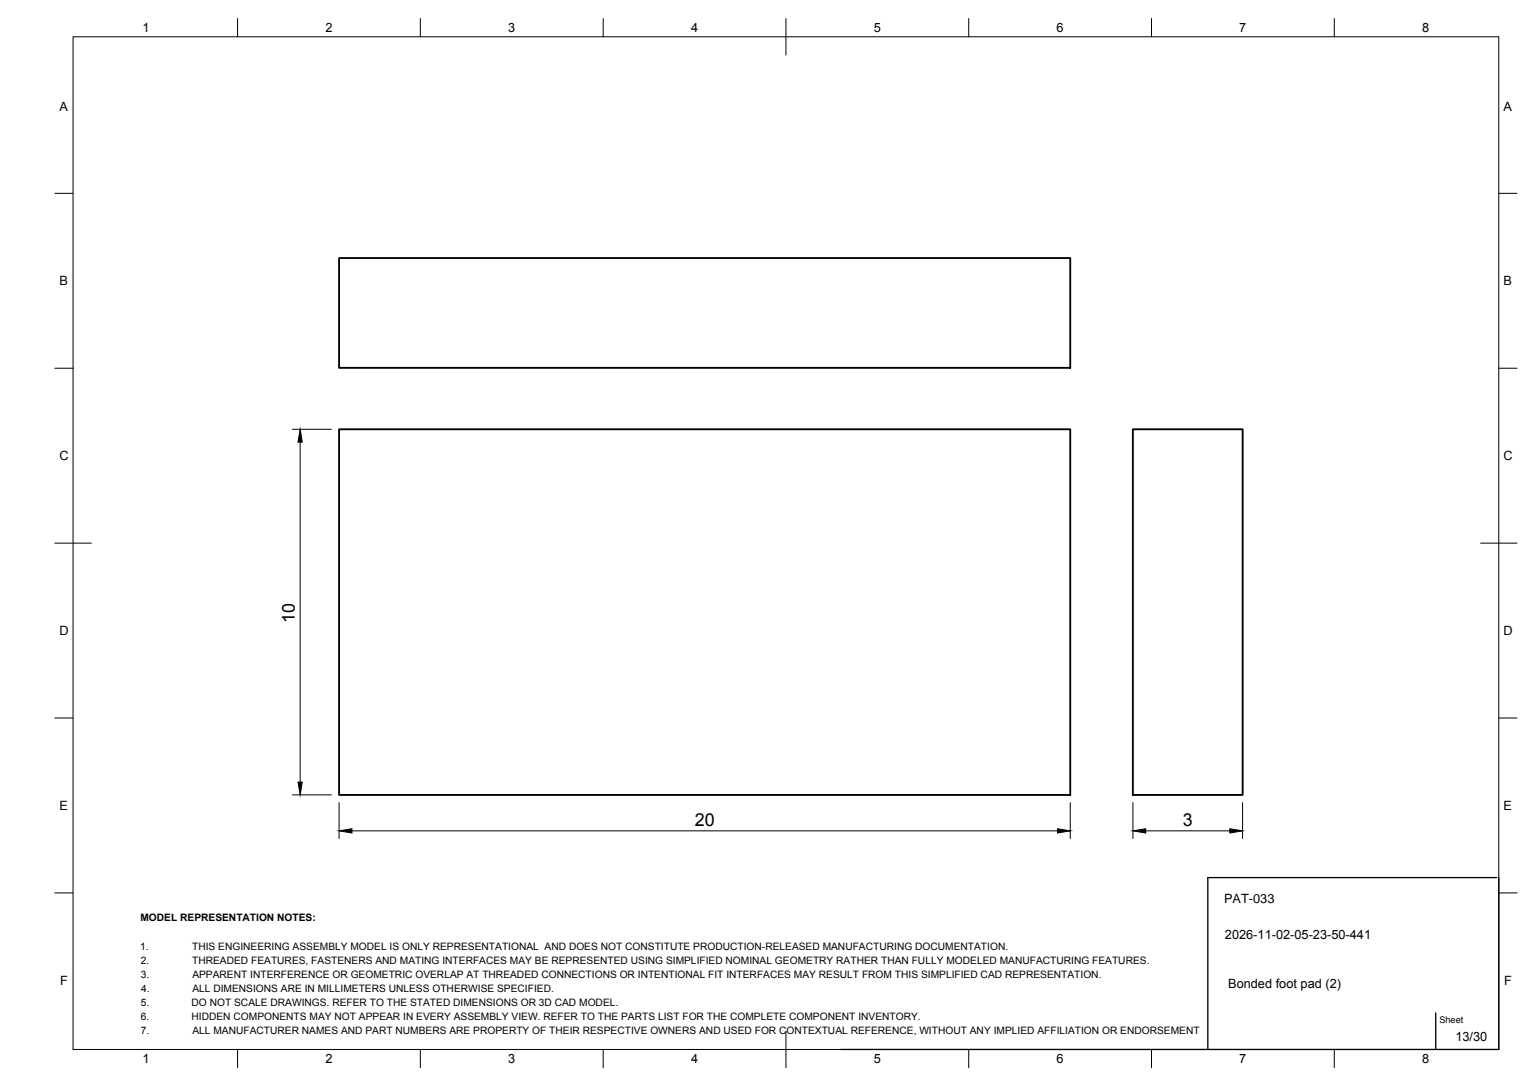
ISO-10303-21;
HEADER;
/* Generated by software containing ST-Developer
 * from STEP Tools, Inc. (www.steptools.com) 
 */

FILE_DESCRIPTION(
/* description */ ('Dual-rail gantry carriage'),
/* implementation_level */ '2;1');

FILE_NAME(
/* name */ 'Bonded foot pad (2).step',
/* time_stamp */ '2026-10-27T10:49:15-07:00',
/* author */ (''),
/* organization */ (''),
/* preprocessor_version */ 'ST-DEVELOPER v20.2',
/* originating_system */ 'Autodesk Translation Framework v15.17.0.0',
/* authorisation */ '');

FILE_SCHEMA (('AUTOMOTIVE_DESIGN { 1 0 10303 214 3 1 1 }'));
ENDSEC;

DATA;
#10=MECHANICAL_DESIGN_GEOMETRIC_PRESENTATION_REPRESENTATION('',(#593),#12804);
#531=SHAPE_REPRESENTATION_RELATIONSHIP('SRR','None',#13009,#562);
#562=ADVANCED_BREP_SHAPE_REPRESENTATION('',(#624),#12779);
#593=STYLED_ITEM('',(#13240),#624);
#624=MANIFOLD_SOLID_BREP('Body1',#7371);
#812=PLANE('',#7860);
#813=PLANE('',#7861);
#814=PLANE('',#7862);
#815=PLANE('',#7863);
#816=PLANE('',#7864);
#817=PLANE('',#7865);
#1116=FACE_OUTER_BOUND('',#1545,.T.);
#1117=FACE_OUTER_BOUND('',#1546,.T.);
#1118=FACE_OUTER_BOUND('',#1547,.T.);
#1119=FACE_OUTER_BOUND('',#1548,.T.);
#1120=FACE_OUTER_BOUND('',#1549,.T.);
#1121=FACE_OUTER_BOUND('',#1550,.T.);
#1545=EDGE_LOOP('',(#5379,#5380,#5381,#5382));
#1546=EDGE_LOOP('',(#5383,#5384,#5385,#5386));
#1547=EDGE_LOOP('',(#5387,#5388,#5389,#5390));
#1548=EDGE_LOOP('',(#5391,#5392,#5393,#5394));
#1549=EDGE_LOOP('',(#5395,#5396,#5397,#5398));
#1550=EDGE_LOOP('',(#5399,#5400,#5401,#5402));
#2064=LINE('',#11030,#2773);
#2065=LINE('',#11032,#2774);
#2066=LINE('',#11034,#2775);
#2067=LINE('',#11035,#2776);
#2068=LINE('',#11038,#2777);
#2069=LINE('',#11040,#2778);
#2070=LINE('',#11041,#2779);
#2071=LINE('',#11044,#2780);
#2072=LINE('',#11046,#2781);
#2073=LINE('',#11047,#2782);
#2074=LINE('',#11049,#2783);
#2075=LINE('',#11050,#2784);
#2773=VECTOR('',#8843,1.);
#2774=VECTOR('',#8844,1.);
#2775=VECTOR('',#8845,1.);
#2776=VECTOR('',#8846,1.);
#2777=VECTOR('',#8849,1.);
#2778=VECTOR('',#8850,1.);
#2779=VECTOR('',#8851,1.);
#2780=VECTOR('',#8854,1.);
#2781=VECTOR('',#8855,1.);
#2782=VECTOR('',#8856,1.);
#2783=VECTOR('',#8859,1.);
#2784=VECTOR('',#8860,1.);
#3670=VERTEX_POINT('',#11028);
#3671=VERTEX_POINT('',#11029);
#3672=VERTEX_POINT('',#11031);
#3673=VERTEX_POINT('',#11033);
#3674=VERTEX_POINT('',#11037);
#3675=VERTEX_POINT('',#11039);
#3676=VERTEX_POINT('',#11043);
#3677=VERTEX_POINT('',#11045);
#4312=EDGE_CURVE('',#3670,#3671,#2064,.T.);
#4313=EDGE_CURVE('',#3671,#3672,#2065,.T.);
#4314=EDGE_CURVE('',#3673,#3672,#2066,.T.);
#4315=EDGE_CURVE('',#3670,#3673,#2067,.T.);
#4316=EDGE_CURVE('',#3674,#3670,#2068,.T.);
#4317=EDGE_CURVE('',#3675,#3673,#2069,.T.);
#4318=EDGE_CURVE('',#3674,#3675,#2070,.T.);
#4319=EDGE_CURVE('',#3676,#3674,#2071,.T.);
#4320=EDGE_CURVE('',#3677,#3675,#2072,.T.);
#4321=EDGE_CURVE('',#3676,#3677,#2073,.T.);
#4322=EDGE_CURVE('',#3671,#3676,#2074,.T.);
#4323=EDGE_CURVE('',#3672,#3677,#2075,.T.);
#5379=ORIENTED_EDGE('',*,*,#4312,.T.);
#5380=ORIENTED_EDGE('',*,*,#4313,.T.);
#5381=ORIENTED_EDGE('',*,*,#4314,.F.);
#5382=ORIENTED_EDGE('',*,*,#4315,.F.);
#5383=ORIENTED_EDGE('',*,*,#4316,.T.);
#5384=ORIENTED_EDGE('',*,*,#4315,.T.);
#5385=ORIENTED_EDGE('',*,*,#4317,.F.);
#5386=ORIENTED_EDGE('',*,*,#4318,.F.);
#5387=ORIENTED_EDGE('',*,*,#4319,.T.);
#5388=ORIENTED_EDGE('',*,*,#4318,.T.);
#5389=ORIENTED_EDGE('',*,*,#4320,.F.);
#5390=ORIENTED_EDGE('',*,*,#4321,.F.);
#5391=ORIENTED_EDGE('',*,*,#4322,.T.);
#5392=ORIENTED_EDGE('',*,*,#4321,.T.);
#5393=ORIENTED_EDGE('',*,*,#4323,.F.);
#5394=ORIENTED_EDGE('',*,*,#4313,.F.);
#5395=ORIENTED_EDGE('',*,*,#4323,.T.);
#5396=ORIENTED_EDGE('',*,*,#4320,.T.);
#5397=ORIENTED_EDGE('',*,*,#4317,.T.);
#5398=ORIENTED_EDGE('',*,*,#4314,.T.);
#5399=ORIENTED_EDGE('',*,*,#4322,.F.);
#5400=ORIENTED_EDGE('',*,*,#4312,.F.);
#5401=ORIENTED_EDGE('',*,*,#4316,.F.);
#5402=ORIENTED_EDGE('',*,*,#4319,.F.);
#7042=ADVANCED_FACE('',(#1116),#812,.T.);
#7043=ADVANCED_FACE('',(#1117),#813,.T.);
#7044=ADVANCED_FACE('',(#1118),#814,.T.);
#7045=ADVANCED_FACE('',(#1119),#815,.T.);
#7046=ADVANCED_FACE('',(#1120),#816,.T.);
#7047=ADVANCED_FACE('',(#1121),#817,.F.);
#7371=CLOSED_SHELL('',(#7042,#7043,#7044,#7045,#7046,#7047));
#7859=AXIS2_PLACEMENT_3D('',#11026,#8839,#8840);
#7860=AXIS2_PLACEMENT_3D('',#11027,#8841,#8842);
#7861=AXIS2_PLACEMENT_3D('',#11036,#8847,#8848);
#7862=AXIS2_PLACEMENT_3D('',#11042,#8852,#8853);
#7863=AXIS2_PLACEMENT_3D('',#11048,#8857,#8858);
#7864=AXIS2_PLACEMENT_3D('',#11051,#8861,#8862);
#7865=AXIS2_PLACEMENT_3D('',#11052,#8863,#8864);
#8839=DIRECTION('axis',(0.,0.,1.));
#8840=DIRECTION('refdir',(1.,0.,0.));
#8841=DIRECTION('center_axis',(0.,1.,0.));
#8842=DIRECTION('ref_axis',(-1.,0.,0.));
#8843=DIRECTION('',(-1.,0.,0.));
#8844=DIRECTION('',(0.,0.,1.));
#8845=DIRECTION('',(-1.,0.,0.));
#8846=DIRECTION('',(0.,0.,1.));
#8847=DIRECTION('center_axis',(1.,0.,0.));
#8848=DIRECTION('ref_axis',(0.,1.,0.));
#8849=DIRECTION('',(0.,1.,0.));
#8850=DIRECTION('',(0.,1.,0.));
#8851=DIRECTION('',(0.,0.,1.));
#8852=DIRECTION('center_axis',(0.,-1.,0.));
#8853=DIRECTION('ref_axis',(1.,0.,0.));
#8854=DIRECTION('',(1.,0.,0.));
#8855=DIRECTION('',(1.,0.,0.));
#8856=DIRECTION('',(0.,0.,1.));
#8857=DIRECTION('center_axis',(-1.,0.,0.));
#8858=DIRECTION('ref_axis',(0.,-1.,0.));
#8859=DIRECTION('',(0.,-1.,0.));
#8860=DIRECTION('',(0.,-1.,0.));
#8861=DIRECTION('center_axis',(0.,0.,1.));
#8862=DIRECTION('ref_axis',(1.,0.,0.));
#8863=DIRECTION('center_axis',(0.,0.,1.));
#8864=DIRECTION('ref_axis',(1.,0.,0.));
#11026=CARTESIAN_POINT('',(0.,0.,0.));
#11027=CARTESIAN_POINT('Origin',(40.,-11.5,-1.1));
#11028=CARTESIAN_POINT('',(40.,-11.5,-1.1));
#11029=CARTESIAN_POINT('',(38.,-11.5,-1.1));
#11030=CARTESIAN_POINT('',(40.,-11.5,-1.1));
#11031=CARTESIAN_POINT('',(38.,-11.5,-0.8));
#11032=CARTESIAN_POINT('',(38.,-11.5,-1.1));
#11033=CARTESIAN_POINT('',(40.,-11.5,-0.8));
#11034=CARTESIAN_POINT('',(40.,-11.5,-0.8));
#11035=CARTESIAN_POINT('',(40.,-11.5,-1.1));
#11036=CARTESIAN_POINT('Origin',(40.,-12.5,-1.1));
#11037=CARTESIAN_POINT('',(40.,-12.5,-1.1));
#11038=CARTESIAN_POINT('',(40.,-12.5,-1.1));
#11039=CARTESIAN_POINT('',(40.,-12.5,-0.8));
#11040=CARTESIAN_POINT('',(40.,-12.5,-0.8));
#11041=CARTESIAN_POINT('',(40.,-12.5,-1.1));
#11042=CARTESIAN_POINT('Origin',(38.,-12.5,-1.1));
#11043=CARTESIAN_POINT('',(38.,-12.5,-1.1));
#11044=CARTESIAN_POINT('',(38.,-12.5,-1.1));
#11045=CARTESIAN_POINT('',(38.,-12.5,-0.8));
#11046=CARTESIAN_POINT('',(38.,-12.5,-0.8));
#11047=CARTESIAN_POINT('',(38.,-12.5,-1.1));
#11048=CARTESIAN_POINT('Origin',(38.,-11.5,-1.1));
#11049=CARTESIAN_POINT('',(38.,-11.5,-1.1));
#11050=CARTESIAN_POINT('',(38.,-11.5,-0.8));
#11051=CARTESIAN_POINT('Origin',(39.,-12.,-0.8));
#11052=CARTESIAN_POINT('Origin',(39.,-12.,-1.1));
#12743=UNCERTAINTY_MEASURE_WITH_UNIT(LENGTH_MEASURE(0.001),#12805,
'DISTANCE_ACCURACY_VALUE',
'Maximum model space distance between geometric entities at asserted c
onnectivities');
#12768=UNCERTAINTY_MEASURE_WITH_UNIT(LENGTH_MEASURE(0.001),#12805,
'DISTANCE_ACCURACY_VALUE',
'Maximum model space distance between geometric entities at asserted c
onnectivities');
#12779=(
GEOMETRIC_REPRESENTATION_CONTEXT(3)
GLOBAL_UNCERTAINTY_ASSIGNED_CONTEXT((#12743))
GLOBAL_UNIT_ASSIGNED_CONTEXT((#12805,#12807,#12808))
REPRESENTATION_CONTEXT('','3D')
);
#12804=(
GEOMETRIC_REPRESENTATION_CONTEXT(3)
GLOBAL_UNCERTAINTY_ASSIGNED_CONTEXT((#12768))
GLOBAL_UNIT_ASSIGNED_CONTEXT((#12805,#12807,#12808))
REPRESENTATION_CONTEXT('','3D')
);
#12805=(
LENGTH_UNIT()
NAMED_UNIT(*)
SI_UNIT(.CENTI.,.METRE.)
);
#12807=(
NAMED_UNIT(*)
PLANE_ANGLE_UNIT()
SI_UNIT($,.RADIAN.)
);
#12808=(
NAMED_UNIT(*)
SI_UNIT($,.STERADIAN.)
SOLID_ANGLE_UNIT()
);
#12819=SHAPE_DEFINITION_REPRESENTATION(#12854,#13009);
#12854=PRODUCT_DEFINITION_SHAPE('',$,#13045);
#13009=SHAPE_REPRESENTATION('',(#7859),#12779);
#13034=PRODUCT_DEFINITION_CONTEXT('part definition',#13141,'design');
#13045=PRODUCT_DEFINITION('Bonded foot pad (2)','Bonded foot pad (2)',#13080,
#13034);
#13080=PRODUCT_DEFINITION_FORMATION('',$,#13153);
#13141=APPLICATION_CONTEXT(
'Core Data for Automotive Mechanical Design Process');
#13142=PRODUCT_CONTEXT('part definition',#13141,'mechanical');
#13153=PRODUCT('Bonded foot pad (2)','Bonded foot pad (2)',
'Bonded foot pad (2)',(#13142));
#13234=COLOUR_RGB('Sky Blue',0.24,0.69,0.87);
#13235=FILL_AREA_STYLE_COLOUR('',#13234);
#13236=FILL_AREA_STYLE('',(#13235));
#13237=SURFACE_STYLE_FILL_AREA(#13236);
#13238=SURFACE_SIDE_STYLE('',(#13237));
#13239=SURFACE_STYLE_USAGE(.BOTH.,#13238);
#13240=PRESENTATION_STYLE_ASSIGNMENT((#13239));
ENDSEC;
END-ISO-10303-21;
